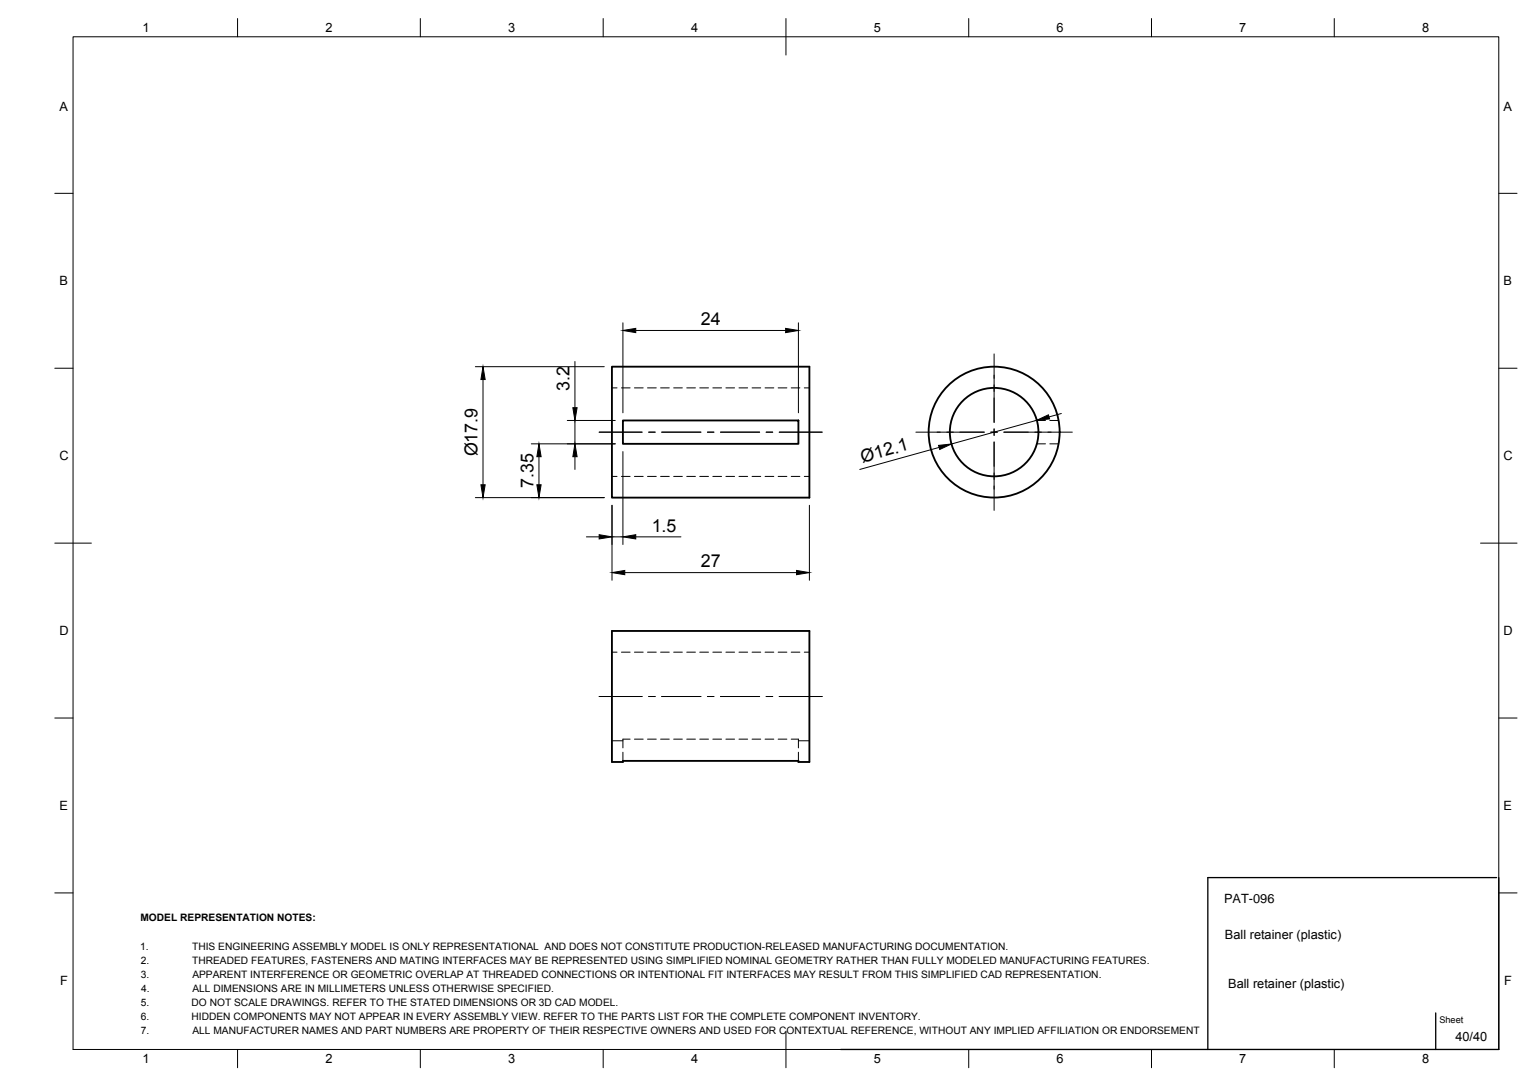
ISO-10303-21;
HEADER;
/* Generated by software containing ST-Developer
 * from STEP Tools, Inc. (www.steptools.com) 
 */

FILE_DESCRIPTION(
/* description */ ('PAT-096'),
/* implementation_level */ '2;1');

FILE_NAME(
/* name */ 'Ball retainer (plastic).step',
/* time_stamp */ '2026-10-29T17:03:14-07:00',
/* author */ (''),
/* organization */ (''),
/* preprocessor_version */ 'ST-DEVELOPER v20.2',
/* originating_system */ 'Autodesk Translation Framework v15.17.0.0',
/* authorisation */ '');

FILE_SCHEMA (('AUTOMOTIVE_DESIGN { 1 0 10303 214 3 1 1 }'));
ENDSEC;

DATA;
#10=MECHANICAL_DESIGN_GEOMETRIC_PRESENTATION_REPRESENTATION('',(#432),#10650);
#362=SHAPE_REPRESENTATION_RELATIONSHIP('SRR','None',#10827,#393);
#393=ADVANCED_BREP_SHAPE_REPRESENTATION('',(#469),#10645);
#432=STYLED_ITEM('',(#11057),#469);
#469=MANIFOLD_SOLID_BREP('Body1',#5567);
#593=FACE_BOUND('',#1544,.T.);
#594=FACE_BOUND('',#1546,.T.);
#595=FACE_BOUND('',#1548,.T.);
#596=FACE_BOUND('',#1550,.T.);
#763=PLANE('',#6536);
#764=PLANE('',#6539);
#765=PLANE('',#6540);
#766=PLANE('',#6543);
#767=PLANE('',#6544);
#768=PLANE('',#6549);
#1083=FACE_OUTER_BOUND('',#1539,.T.);
#1084=FACE_OUTER_BOUND('',#1540,.T.);
#1085=FACE_OUTER_BOUND('',#1541,.T.);
#1086=FACE_OUTER_BOUND('',#1542,.T.);
#1087=FACE_OUTER_BOUND('',#1543,.T.);
#1088=FACE_OUTER_BOUND('',#1545,.T.);
#1089=FACE_OUTER_BOUND('',#1547,.T.);
#1090=FACE_OUTER_BOUND('',#1549,.T.);
#1539=EDGE_LOOP('',(#4899,#4900,#4901,#4902));
#1540=EDGE_LOOP('',(#4903,#4904,#4905,#4906));
#1541=EDGE_LOOP('',(#4907,#4908,#4909,#4910));
#1542=EDGE_LOOP('',(#4911,#4912,#4913,#4914));
#1543=EDGE_LOOP('',(#4915));
#1544=EDGE_LOOP('',(#4916));
#1545=EDGE_LOOP('',(#4917,#4918,#4919,#4920));
#1546=EDGE_LOOP('',(#4921,#4922,#4923,#4924));
#1547=EDGE_LOOP('',(#4925));
#1548=EDGE_LOOP('',(#4926));
#1549=EDGE_LOOP('',(#4927,#4928,#4929,#4930));
#1550=EDGE_LOOP('',(#4931,#4932,#4933,#4934));
#1876=LINE('',#10332,#2205);
#1877=LINE('',#10335,#2206);
#1878=LINE('',#10338,#2207);
#1879=LINE('',#10340,#2208);
#1880=LINE('',#10341,#2209);
#1881=LINE('',#10347,#2210);
#1882=LINE('',#10349,#2211);
#1883=LINE('',#10350,#2212);
#1884=LINE('',#10359,#2213);
#1885=LINE('',#10364,#2214);
#2205=VECTOR('',#8192,1.);
#2206=VECTOR('',#8195,1.);
#2207=VECTOR('',#8198,1.);
#2208=VECTOR('',#8199,1.);
#2209=VECTOR('',#8200,1.);
#2210=VECTOR('',#8207,1.);
#2211=VECTOR('',#8210,1.);
#2212=VECTOR('',#8211,1.);
#2213=VECTOR('',#8222,0.895);
#2214=VECTOR('',#8229,0.605);
#2545=CIRCLE('',#6537,0.895);
#2546=CIRCLE('',#6538,0.605);
#2547=CIRCLE('',#6541,0.895);
#2548=CIRCLE('',#6542,0.605);
#2549=CIRCLE('',#6545,0.895);
#2550=CIRCLE('',#6546,0.605);
#2551=CIRCLE('',#6548,0.895);
#2552=CIRCLE('',#6550,0.605);
#2979=VERTEX_POINT('',#10328);
#2980=VERTEX_POINT('',#10329);
#2981=VERTEX_POINT('',#10331);
#2982=VERTEX_POINT('',#10333);
#2983=VERTEX_POINT('',#10337);
#2984=VERTEX_POINT('',#10339);
#2985=VERTEX_POINT('',#10343);
#2986=VERTEX_POINT('',#10345);
#2987=VERTEX_POINT('',#10352);
#2988=VERTEX_POINT('',#10354);
#2989=VERTEX_POINT('',#10357);
#2990=VERTEX_POINT('',#10361);
#3628=EDGE_CURVE('',#2979,#2980,#2545,.T.);
#3629=EDGE_CURVE('',#2981,#2979,#1876,.T.);
#3630=EDGE_CURVE('',#2982,#2981,#2546,.T.);
#3631=EDGE_CURVE('',#2980,#2982,#1877,.T.);
#3632=EDGE_CURVE('',#2980,#2983,#1878,.T.);
#3633=EDGE_CURVE('',#2984,#2982,#1879,.T.);
#3634=EDGE_CURVE('',#2984,#2983,#1880,.T.);
#3635=EDGE_CURVE('',#2983,#2985,#2547,.T.);
#3636=EDGE_CURVE('',#2986,#2984,#2548,.T.);
#3637=EDGE_CURVE('',#2985,#2986,#1881,.T.);
#3638=EDGE_CURVE('',#2985,#2979,#1882,.T.);
#3639=EDGE_CURVE('',#2981,#2986,#1883,.T.);
#3640=EDGE_CURVE('',#2987,#2987,#2549,.T.);
#3641=EDGE_CURVE('',#2988,#2988,#2550,.T.);
#3642=EDGE_CURVE('',#2989,#2989,#2551,.T.);
#3643=EDGE_CURVE('',#2989,#2987,#1884,.T.);
#3644=EDGE_CURVE('',#2990,#2990,#2552,.T.);
#3645=EDGE_CURVE('',#2990,#2988,#1885,.T.);
#4899=ORIENTED_EDGE('',*,*,#3628,.F.);
#4900=ORIENTED_EDGE('',*,*,#3629,.F.);
#4901=ORIENTED_EDGE('',*,*,#3630,.F.);
#4902=ORIENTED_EDGE('',*,*,#3631,.F.);
#4903=ORIENTED_EDGE('',*,*,#3632,.F.);
#4904=ORIENTED_EDGE('',*,*,#3631,.T.);
#4905=ORIENTED_EDGE('',*,*,#3633,.F.);
#4906=ORIENTED_EDGE('',*,*,#3634,.T.);
#4907=ORIENTED_EDGE('',*,*,#3635,.F.);
#4908=ORIENTED_EDGE('',*,*,#3634,.F.);
#4909=ORIENTED_EDGE('',*,*,#3636,.F.);
#4910=ORIENTED_EDGE('',*,*,#3637,.F.);
#4911=ORIENTED_EDGE('',*,*,#3638,.F.);
#4912=ORIENTED_EDGE('',*,*,#3637,.T.);
#4913=ORIENTED_EDGE('',*,*,#3639,.F.);
#4914=ORIENTED_EDGE('',*,*,#3629,.T.);
#4915=ORIENTED_EDGE('',*,*,#3640,.F.);
#4916=ORIENTED_EDGE('',*,*,#3641,.T.);
#4917=ORIENTED_EDGE('',*,*,#3642,.F.);
#4918=ORIENTED_EDGE('',*,*,#3643,.T.);
#4919=ORIENTED_EDGE('',*,*,#3640,.T.);
#4920=ORIENTED_EDGE('',*,*,#3643,.F.);
#4921=ORIENTED_EDGE('',*,*,#3635,.T.);
#4922=ORIENTED_EDGE('',*,*,#3638,.T.);
#4923=ORIENTED_EDGE('',*,*,#3628,.T.);
#4924=ORIENTED_EDGE('',*,*,#3632,.T.);
#4925=ORIENTED_EDGE('',*,*,#3642,.T.);
#4926=ORIENTED_EDGE('',*,*,#3644,.F.);
#4927=ORIENTED_EDGE('',*,*,#3644,.T.);
#4928=ORIENTED_EDGE('',*,*,#3645,.T.);
#4929=ORIENTED_EDGE('',*,*,#3641,.F.);
#4930=ORIENTED_EDGE('',*,*,#3645,.F.);
#4931=ORIENTED_EDGE('',*,*,#3636,.T.);
#4932=ORIENTED_EDGE('',*,*,#3633,.T.);
#4933=ORIENTED_EDGE('',*,*,#3630,.T.);
#4934=ORIENTED_EDGE('',*,*,#3639,.T.);
#5182=CYLINDRICAL_SURFACE('',#6547,0.895);
#5183=CYLINDRICAL_SURFACE('',#6551,0.605);
#5488=ADVANCED_FACE('',(#1083),#763,.F.);
#5489=ADVANCED_FACE('',(#1084),#764,.F.);
#5490=ADVANCED_FACE('',(#1085),#765,.F.);
#5491=ADVANCED_FACE('',(#1086),#766,.F.);
#5492=ADVANCED_FACE('',(#1087,#593),#767,.T.);
#5493=ADVANCED_FACE('',(#1088,#594),#5182,.T.);
#5494=ADVANCED_FACE('',(#1089,#595),#768,.T.);
#5495=ADVANCED_FACE('',(#1090,#596),#5183,.F.);
#5567=CLOSED_SHELL('',(#5488,#5489,#5490,#5491,#5492,#5493,#5494,#5495));
#6535=AXIS2_PLACEMENT_3D('',#10326,#8186,#8187);
#6536=AXIS2_PLACEMENT_3D('',#10327,#8188,#8189);
#6537=AXIS2_PLACEMENT_3D('',#10330,#8190,#8191);
#6538=AXIS2_PLACEMENT_3D('',#10334,#8193,#8194);
#6539=AXIS2_PLACEMENT_3D('',#10336,#8196,#8197);
#6540=AXIS2_PLACEMENT_3D('',#10342,#8201,#8202);
#6541=AXIS2_PLACEMENT_3D('',#10344,#8203,#8204);
#6542=AXIS2_PLACEMENT_3D('',#10346,#8205,#8206);
#6543=AXIS2_PLACEMENT_3D('',#10348,#8208,#8209);
#6544=AXIS2_PLACEMENT_3D('',#10351,#8212,#8213);
#6545=AXIS2_PLACEMENT_3D('',#10353,#8214,#8215);
#6546=AXIS2_PLACEMENT_3D('',#10355,#8216,#8217);
#6547=AXIS2_PLACEMENT_3D('',#10356,#8218,#8219);
#6548=AXIS2_PLACEMENT_3D('',#10358,#8220,#8221);
#6549=AXIS2_PLACEMENT_3D('',#10360,#8223,#8224);
#6550=AXIS2_PLACEMENT_3D('',#10362,#8225,#8226);
#6551=AXIS2_PLACEMENT_3D('',#10363,#8227,#8228);
#8186=DIRECTION('axis',(0.,0.,1.));
#8187=DIRECTION('refdir',(1.,0.,0.));
#8188=DIRECTION('center_axis',(0.,1.,0.));
#8189=DIRECTION('ref_axis',(0.,0.,1.));
#8190=DIRECTION('center_axis',(0.,1.,0.));
#8191=DIRECTION('ref_axis',(1.,0.,0.));
#8192=DIRECTION('',(1.,0.,0.));
#8193=DIRECTION('center_axis',(0.,-1.,0.));
#8194=DIRECTION('ref_axis',(1.,0.,0.));
#8195=DIRECTION('',(-1.,0.,0.));
#8196=DIRECTION('center_axis',(0.,0.,-1.));
#8197=DIRECTION('ref_axis',(-1.,0.,0.));
#8198=DIRECTION('',(0.,-1.,0.));
#8199=DIRECTION('',(0.,1.,0.));
#8200=DIRECTION('',(1.,0.,0.));
#8201=DIRECTION('center_axis',(0.,-1.,0.));
#8202=DIRECTION('ref_axis',(0.,0.,-1.));
#8203=DIRECTION('center_axis',(0.,-1.,0.));
#8204=DIRECTION('ref_axis',(1.,0.,0.));
#8205=DIRECTION('center_axis',(0.,1.,0.));
#8206=DIRECTION('ref_axis',(1.,0.,0.));
#8207=DIRECTION('',(-1.,0.,0.));
#8208=DIRECTION('center_axis',(0.,0.,1.));
#8209=DIRECTION('ref_axis',(1.,0.,0.));
#8210=DIRECTION('',(0.,1.,0.));
#8211=DIRECTION('',(0.,-1.,0.));
#8212=DIRECTION('center_axis',(0.,1.,0.));
#8213=DIRECTION('ref_axis',(0.,0.,1.));
#8214=DIRECTION('center_axis',(0.,-1.,0.));
#8215=DIRECTION('ref_axis',(1.,0.,0.));
#8216=DIRECTION('center_axis',(0.,-1.,0.));
#8217=DIRECTION('ref_axis',(1.,0.,0.));
#8218=DIRECTION('center_axis',(0.,-1.,0.));
#8219=DIRECTION('ref_axis',(1.,0.,0.));
#8220=DIRECTION('center_axis',(0.,-1.,0.));
#8221=DIRECTION('ref_axis',(1.,0.,0.));
#8222=DIRECTION('',(0.,1.,0.));
#8223=DIRECTION('center_axis',(0.,-1.,0.));
#8224=DIRECTION('ref_axis',(0.,0.,-1.));
#8225=DIRECTION('center_axis',(0.,-1.,0.));
#8226=DIRECTION('ref_axis',(1.,0.,0.));
#8227=DIRECTION('center_axis',(0.,-1.,0.));
#8228=DIRECTION('ref_axis',(1.,0.,0.));
#8229=DIRECTION('',(0.,1.,0.));
#10326=CARTESIAN_POINT('',(0.,0.,0.));
#10327=CARTESIAN_POINT('Origin',(0.75,1.2,0.));
#10328=CARTESIAN_POINT('',(0.880582193778639,1.2,0.16));
#10329=CARTESIAN_POINT('',(0.880582193778639,1.2,-0.16));
#10330=CARTESIAN_POINT('Origin',(0.,1.2,0.));
#10331=CARTESIAN_POINT('',(0.583459510163302,1.2,0.16));
#10332=CARTESIAN_POINT('',(0.57,1.2,0.16));
#10333=CARTESIAN_POINT('',(0.583459510163302,1.2,-0.16));
#10334=CARTESIAN_POINT('Origin',(0.,1.2,0.));
#10335=CARTESIAN_POINT('',(0.93,1.2,-0.16));
#10336=CARTESIAN_POINT('Origin',(0.93,0.,-0.16));
#10337=CARTESIAN_POINT('',(0.880582193778639,-1.2,-0.16));
#10338=CARTESIAN_POINT('',(0.880582193778639,0.,-0.16));
#10339=CARTESIAN_POINT('',(0.583459510163302,-1.2,-0.16));
#10340=CARTESIAN_POINT('',(0.583459510163302,0.,-0.16));
#10341=CARTESIAN_POINT('',(0.93,-1.2,-0.16));
#10342=CARTESIAN_POINT('Origin',(0.75,-1.2,0.));
#10343=CARTESIAN_POINT('',(0.880582193778639,-1.2,0.16));
#10344=CARTESIAN_POINT('Origin',(0.,-1.2,0.));
#10345=CARTESIAN_POINT('',(0.583459510163302,-1.2,0.16));
#10346=CARTESIAN_POINT('Origin',(0.,-1.2,0.));
#10347=CARTESIAN_POINT('',(0.57,-1.2,0.16));
#10348=CARTESIAN_POINT('Origin',(0.57,0.,0.16));
#10349=CARTESIAN_POINT('',(0.880582193778639,0.,0.16));
#10350=CARTESIAN_POINT('',(0.583459510163302,0.,0.16));
#10351=CARTESIAN_POINT('Origin',(0.895,1.35,0.));
#10352=CARTESIAN_POINT('',(-0.895,1.35,-1.09605888523688E-16));
#10353=CARTESIAN_POINT('Origin',(0.,1.35,0.));
#10354=CARTESIAN_POINT('',(-0.605,1.35,-7.40911313484149E-17));
#10355=CARTESIAN_POINT('Origin',(0.,1.35,0.));
#10356=CARTESIAN_POINT('Origin',(0.,0.,0.));
#10357=CARTESIAN_POINT('',(-0.895,-1.35,-1.09605888523688E-16));
#10358=CARTESIAN_POINT('Origin',(0.,-1.35,0.));
#10359=CARTESIAN_POINT('',(-0.895,0.,-1.09605888523688E-16));
#10360=CARTESIAN_POINT('Origin',(0.605,-1.35,0.));
#10361=CARTESIAN_POINT('',(-0.605,-1.35,-7.40911313484149E-17));
#10362=CARTESIAN_POINT('Origin',(0.,-1.35,0.));
#10363=CARTESIAN_POINT('Origin',(0.,0.,0.));
#10364=CARTESIAN_POINT('',(-0.605,0.,-7.40911313484149E-17));
#10606=UNCERTAINTY_MEASURE_WITH_UNIT(LENGTH_MEASURE(0.001),#10651,
'DISTANCE_ACCURACY_VALUE',
'Maximum model space distance between geometric entities at asserted c
onnectivities');
#10611=UNCERTAINTY_MEASURE_WITH_UNIT(LENGTH_MEASURE(0.001),#10651,
'DISTANCE_ACCURACY_VALUE',
'Maximum model space distance between geometric entities at asserted c
onnectivities');
#10645=(
GEOMETRIC_REPRESENTATION_CONTEXT(3)
GLOBAL_UNCERTAINTY_ASSIGNED_CONTEXT((#10606))
GLOBAL_UNIT_ASSIGNED_CONTEXT((#10651,#10653,#10654))
REPRESENTATION_CONTEXT('','3D')
);
#10650=(
GEOMETRIC_REPRESENTATION_CONTEXT(3)
GLOBAL_UNCERTAINTY_ASSIGNED_CONTEXT((#10611))
GLOBAL_UNIT_ASSIGNED_CONTEXT((#10651,#10653,#10654))
REPRESENTATION_CONTEXT('','3D')
);
#10651=(
LENGTH_UNIT()
NAMED_UNIT(*)
SI_UNIT(.CENTI.,.METRE.)
);
#10653=(
NAMED_UNIT(*)
PLANE_ANGLE_UNIT()
SI_UNIT($,.RADIAN.)
);
#10654=(
NAMED_UNIT(*)
SI_UNIT($,.STERADIAN.)
SOLID_ANGLE_UNIT()
);
#10688=SHAPE_DEFINITION_REPRESENTATION(#10734,#10827);
#10734=PRODUCT_DEFINITION_SHAPE('',$,#10866);
#10827=SHAPE_REPRESENTATION('',(#6535),#10645);
#10832=PRODUCT_DEFINITION_CONTEXT('part definition',#10948,'design');
#10866=PRODUCT_DEFINITION('Ball retainer (plastic)',
'Ball retainer (plastic)',#10904,#10832);
#10904=PRODUCT_DEFINITION_FORMATION('',$,#10983);
#10948=APPLICATION_CONTEXT(
'Core Data for Automotive Mechanical Design Process');
#10949=PRODUCT_CONTEXT('part definition',#10948,'mechanical');
#10983=PRODUCT('Ball retainer (plastic)','Ball retainer (plastic)',
'Ball retainer (plastic)',(#10949));
#11051=COLOUR_RGB('Sky Blue',0.24,0.69,0.87);
#11052=FILL_AREA_STYLE_COLOUR('',#11051);
#11053=FILL_AREA_STYLE('',(#11052));
#11054=SURFACE_STYLE_FILL_AREA(#11053);
#11055=SURFACE_SIDE_STYLE('',(#11054));
#11056=SURFACE_STYLE_USAGE(.BOTH.,#11055);
#11057=PRESENTATION_STYLE_ASSIGNMENT((#11056));
ENDSEC;
END-ISO-10303-21;
